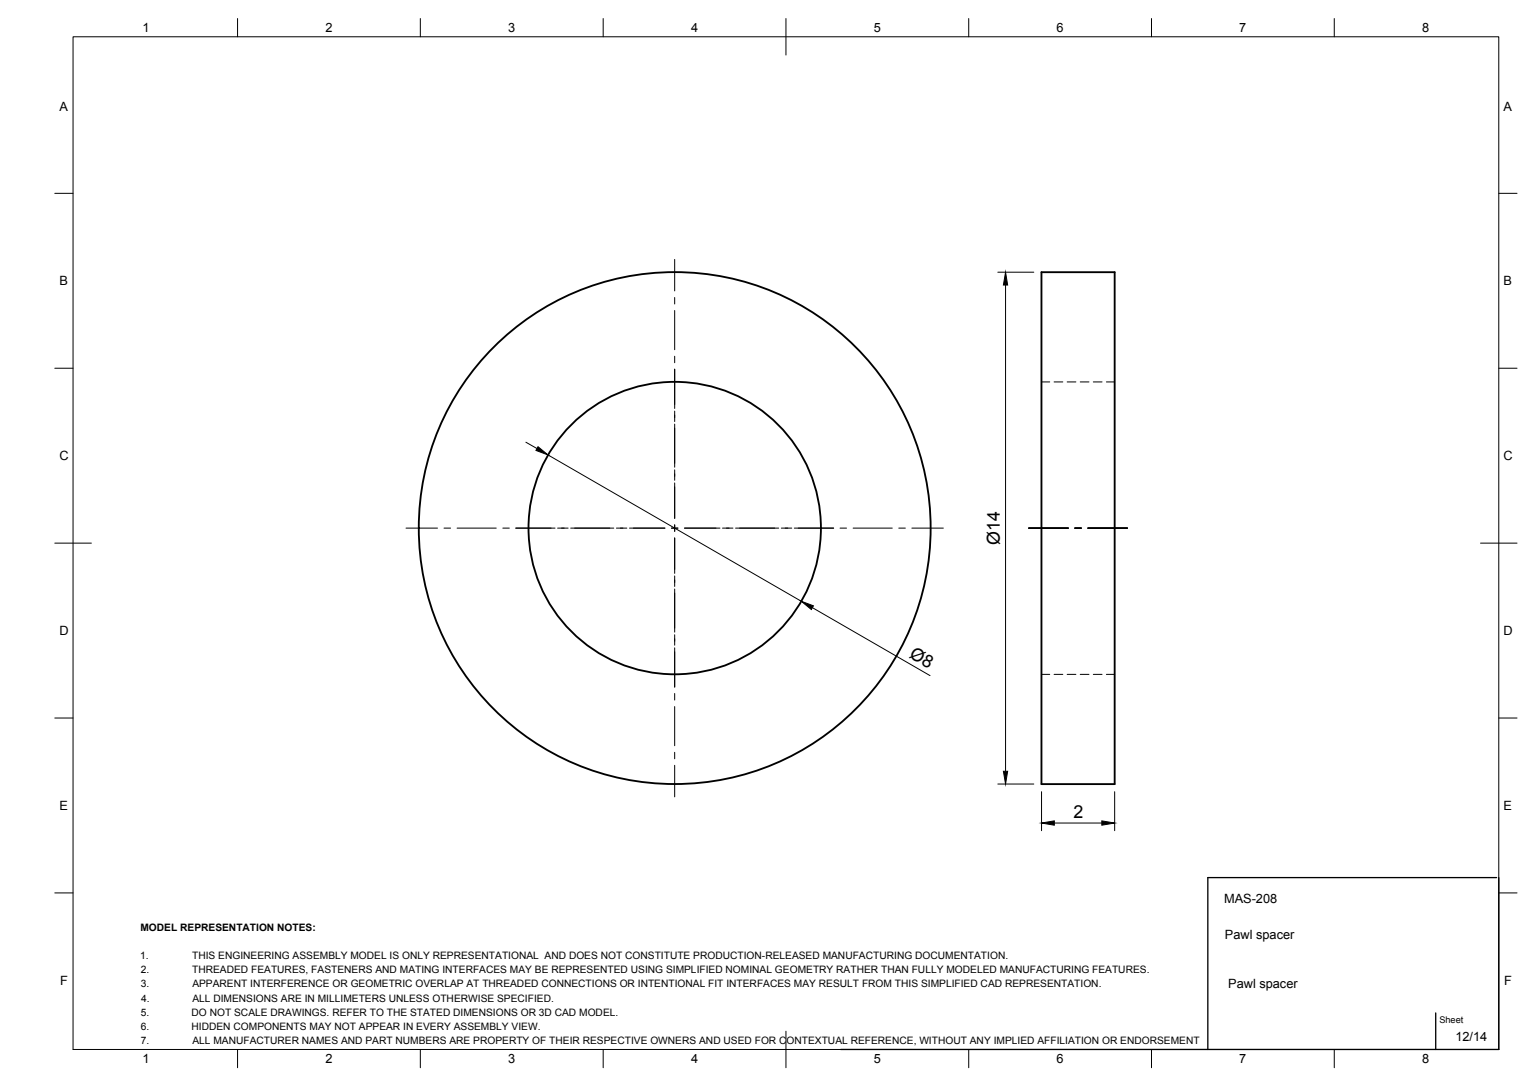
ISO-10303-21;
HEADER;
/* Generated by software containing ST-Developer
 * from STEP Tools, Inc. (www.steptools.com) 
 */

FILE_DESCRIPTION(
/* description */ ('Independent vertical20-tooth ratchet advance with repeated integral-c
ounterweight gravity pawls, swinging drive lever, bronze sleeves and f
ully retained axle stacks.18degpertooth. Native revolutes; geometric c
ycle checking rather than automatic contact/rolling dynamics. Gravity 
closing checked from actual pawl center of mass. Backplate/foot suppor
ts unit. Fits, torque, holding force, wear and life unassigned.'),
/* implementation_level */ '2;1');

FILE_NAME(
/* name */ 'Pawl spacer.step',
/* time_stamp */ '2026-11-09T06:25:53-08:00',
/* author */ (''),
/* organization */ (''),
/* preprocessor_version */ 'ST-DEVELOPER v20.2',
/* originating_system */ 'Autodesk Translation Framework v15.17.0.0',
/* authorisation */ '');

FILE_SCHEMA (('AUTOMOTIVE_DESIGN { 1 0 10303 214 3 1 1 }'));
ENDSEC;

DATA;
#10=MECHANICAL_DESIGN_GEOMETRIC_PRESENTATION_REPRESENTATION('',(#134),#4643);
#106=SHAPE_REPRESENTATION_RELATIONSHIP('SRR','None',#4711,#120);
#120=ADVANCED_BREP_SHAPE_REPRESENTATION('',(#148),#4640);
#134=STYLED_ITEM('',(#4786),#148);
#148=MANIFOLD_SOLID_BREP('Body1',#2670);
#188=FACE_BOUND('',#628,.T.);
#189=FACE_BOUND('',#630,.T.);
#296=PLANE('',#3044);
#297=PLANE('',#3045);
#439=FACE_OUTER_BOUND('',#625,.T.);
#440=FACE_OUTER_BOUND('',#626,.T.);
#441=FACE_OUTER_BOUND('',#627,.T.);
#442=FACE_OUTER_BOUND('',#629,.T.);
#625=EDGE_LOOP('',(#2425,#2426,#2427,#2428));
#626=EDGE_LOOP('',(#2429,#2430,#2431,#2432));
#627=EDGE_LOOP('',(#2433));
#628=EDGE_LOOP('',(#2434));
#629=EDGE_LOOP('',(#2435));
#630=EDGE_LOOP('',(#2436));
#893=LINE('',#4539,#1155);
#894=LINE('',#4545,#1156);
#1155=VECTOR('',#3761,4.);
#1156=VECTOR('',#3768,7.);
#1229=CIRCLE('',#3039,4.);
#1230=CIRCLE('',#3040,4.);
#1231=CIRCLE('',#3042,7.);
#1232=CIRCLE('',#3043,7.);
#1449=VERTEX_POINT('',#4536);
#1450=VERTEX_POINT('',#4538);
#1451=VERTEX_POINT('',#4542);
#1452=VERTEX_POINT('',#4544);
#1777=EDGE_CURVE('',#1449,#1449,#1229,.T.);
#1778=EDGE_CURVE('',#1449,#1450,#893,.T.);
#1779=EDGE_CURVE('',#1450,#1450,#1230,.T.);
#1780=EDGE_CURVE('',#1451,#1451,#1231,.T.);
#1781=EDGE_CURVE('',#1451,#1452,#894,.T.);
#1782=EDGE_CURVE('',#1452,#1452,#1232,.T.);
#2425=ORIENTED_EDGE('',*,*,#1777,.F.);
#2426=ORIENTED_EDGE('',*,*,#1778,.T.);
#2427=ORIENTED_EDGE('',*,*,#1779,.T.);
#2428=ORIENTED_EDGE('',*,*,#1778,.F.);
#2429=ORIENTED_EDGE('',*,*,#1780,.F.);
#2430=ORIENTED_EDGE('',*,*,#1781,.T.);
#2431=ORIENTED_EDGE('',*,*,#1782,.T.);
#2432=ORIENTED_EDGE('',*,*,#1781,.F.);
#2433=ORIENTED_EDGE('',*,*,#1780,.T.);
#2434=ORIENTED_EDGE('',*,*,#1777,.T.);
#2435=ORIENTED_EDGE('',*,*,#1782,.F.);
#2436=ORIENTED_EDGE('',*,*,#1779,.F.);
#2504=CYLINDRICAL_SURFACE('',#3038,4.);
#2505=CYLINDRICAL_SURFACE('',#3041,7.);
#2645=ADVANCED_FACE('',(#439),#2504,.F.);
#2646=ADVANCED_FACE('',(#440),#2505,.T.);
#2647=ADVANCED_FACE('',(#441,#188),#296,.T.);
#2648=ADVANCED_FACE('',(#442,#189),#297,.F.);
#2670=CLOSED_SHELL('',(#2645,#2646,#2647,#2648));
#3037=AXIS2_PLACEMENT_3D('',#4534,#3755,#3756);
#3038=AXIS2_PLACEMENT_3D('',#4535,#3757,#3758);
#3039=AXIS2_PLACEMENT_3D('',#4537,#3759,#3760);
#3040=AXIS2_PLACEMENT_3D('',#4540,#3762,#3763);
#3041=AXIS2_PLACEMENT_3D('',#4541,#3764,#3765);
#3042=AXIS2_PLACEMENT_3D('',#4543,#3766,#3767);
#3043=AXIS2_PLACEMENT_3D('',#4546,#3769,#3770);
#3044=AXIS2_PLACEMENT_3D('',#4547,#3771,#3772);
#3045=AXIS2_PLACEMENT_3D('',#4548,#3773,#3774);
#3755=DIRECTION('axis',(0.,0.,1.));
#3756=DIRECTION('refdir',(1.,0.,0.));
#3757=DIRECTION('center_axis',(0.,0.,1.));
#3758=DIRECTION('ref_axis',(1.,0.,0.));
#3759=DIRECTION('center_axis',(0.,0.,-1.));
#3760=DIRECTION('ref_axis',(1.,0.,0.));
#3761=DIRECTION('',(0.,0.,-1.));
#3762=DIRECTION('center_axis',(0.,0.,-1.));
#3763=DIRECTION('ref_axis',(1.,0.,0.));
#3764=DIRECTION('center_axis',(0.,0.,1.));
#3765=DIRECTION('ref_axis',(1.,0.,0.));
#3766=DIRECTION('center_axis',(0.,0.,1.));
#3767=DIRECTION('ref_axis',(1.,0.,0.));
#3768=DIRECTION('',(0.,0.,-1.));
#3769=DIRECTION('center_axis',(0.,0.,1.));
#3770=DIRECTION('ref_axis',(1.,0.,0.));
#3771=DIRECTION('center_axis',(0.,0.,1.));
#3772=DIRECTION('ref_axis',(1.,0.,0.));
#3773=DIRECTION('center_axis',(0.,0.,1.));
#3774=DIRECTION('ref_axis',(1.,0.,0.));
#4534=CARTESIAN_POINT('',(0.,0.,0.));
#4535=CARTESIAN_POINT('Origin',(0.,0.,0.));
#4536=CARTESIAN_POINT('',(-4.,-4.89858719658941E-16,2.));
#4537=CARTESIAN_POINT('Origin',(0.,0.,2.));
#4538=CARTESIAN_POINT('',(-4.,-4.89858719658941E-16,0.));
#4539=CARTESIAN_POINT('',(-4.,-4.89858719658941E-16,0.));
#4540=CARTESIAN_POINT('Origin',(0.,0.,0.));
#4541=CARTESIAN_POINT('Origin',(0.,0.,0.));
#4542=CARTESIAN_POINT('',(-7.,-8.57252759403147E-16,2.));
#4543=CARTESIAN_POINT('Origin',(0.,0.,2.));
#4544=CARTESIAN_POINT('',(-7.,-8.57252759403147E-16,0.));
#4545=CARTESIAN_POINT('',(-7.,-8.57252759403147E-16,0.));
#4546=CARTESIAN_POINT('Origin',(0.,0.,0.));
#4547=CARTESIAN_POINT('Origin',(0.,0.,2.));
#4548=CARTESIAN_POINT('Origin',(0.,0.,0.));
#4624=UNCERTAINTY_MEASURE_WITH_UNIT(LENGTH_MEASURE(0.01),#4644,
'DISTANCE_ACCURACY_VALUE',
'Maximum model space distance between geometric entities at asserted c
onnectivities');
#4627=UNCERTAINTY_MEASURE_WITH_UNIT(LENGTH_MEASURE(0.01),#4644,
'DISTANCE_ACCURACY_VALUE',
'Maximum model space distance between geometric entities at asserted c
onnectivities');
#4640=(
GEOMETRIC_REPRESENTATION_CONTEXT(3)
GLOBAL_UNCERTAINTY_ASSIGNED_CONTEXT((#4624))
GLOBAL_UNIT_ASSIGNED_CONTEXT((#4644,#4646,#4647))
REPRESENTATION_CONTEXT('','3D')
);
#4643=(
GEOMETRIC_REPRESENTATION_CONTEXT(3)
GLOBAL_UNCERTAINTY_ASSIGNED_CONTEXT((#4627))
GLOBAL_UNIT_ASSIGNED_CONTEXT((#4644,#4646,#4647))
REPRESENTATION_CONTEXT('','3D')
);
#4644=(
LENGTH_UNIT()
NAMED_UNIT(*)
SI_UNIT(.MILLI.,.METRE.)
);
#4646=(
NAMED_UNIT(*)
PLANE_ANGLE_UNIT()
SI_UNIT($,.RADIAN.)
);
#4647=(
NAMED_UNIT(*)
SI_UNIT($,.STERADIAN.)
SOLID_ANGLE_UNIT()
);
#4660=SHAPE_DEFINITION_REPRESENTATION(#4675,#4711);
#4675=PRODUCT_DEFINITION_SHAPE('',$,#4727);
#4711=SHAPE_REPRESENTATION('',(#3037),#4640);
#4714=PRODUCT_DEFINITION_CONTEXT('part definition',#4761,'design');
#4727=PRODUCT_DEFINITION('Pawl spacer','Pawl spacer',#4742,#4714);
#4742=PRODUCT_DEFINITION_FORMATION('',$,#4775);
#4761=APPLICATION_CONTEXT(
'Core Data for Automotive Mechanical Design Process');
#4762=PRODUCT_CONTEXT('part definition',#4761,'mechanical');
#4775=PRODUCT('Pawl spacer','Pawl spacer',$,(#4762));
#4786=PRESENTATION_STYLE_ASSIGNMENT((#4795));
#4795=SURFACE_STYLE_USAGE(.BOTH.,#4804);
#4804=SURFACE_SIDE_STYLE('',(#4813));
#4813=SURFACE_STYLE_FILL_AREA(#4822);
#4822=FILL_AREA_STYLE('Light gray',(#4831));
#4831=FILL_AREA_STYLE_COLOUR('Light gray',#4840);
#4840=COLOUR_RGB('Light gray',0.725490196078431,0.752941176470588,0.792156862745098);
ENDSEC;
END-ISO-10303-21;
